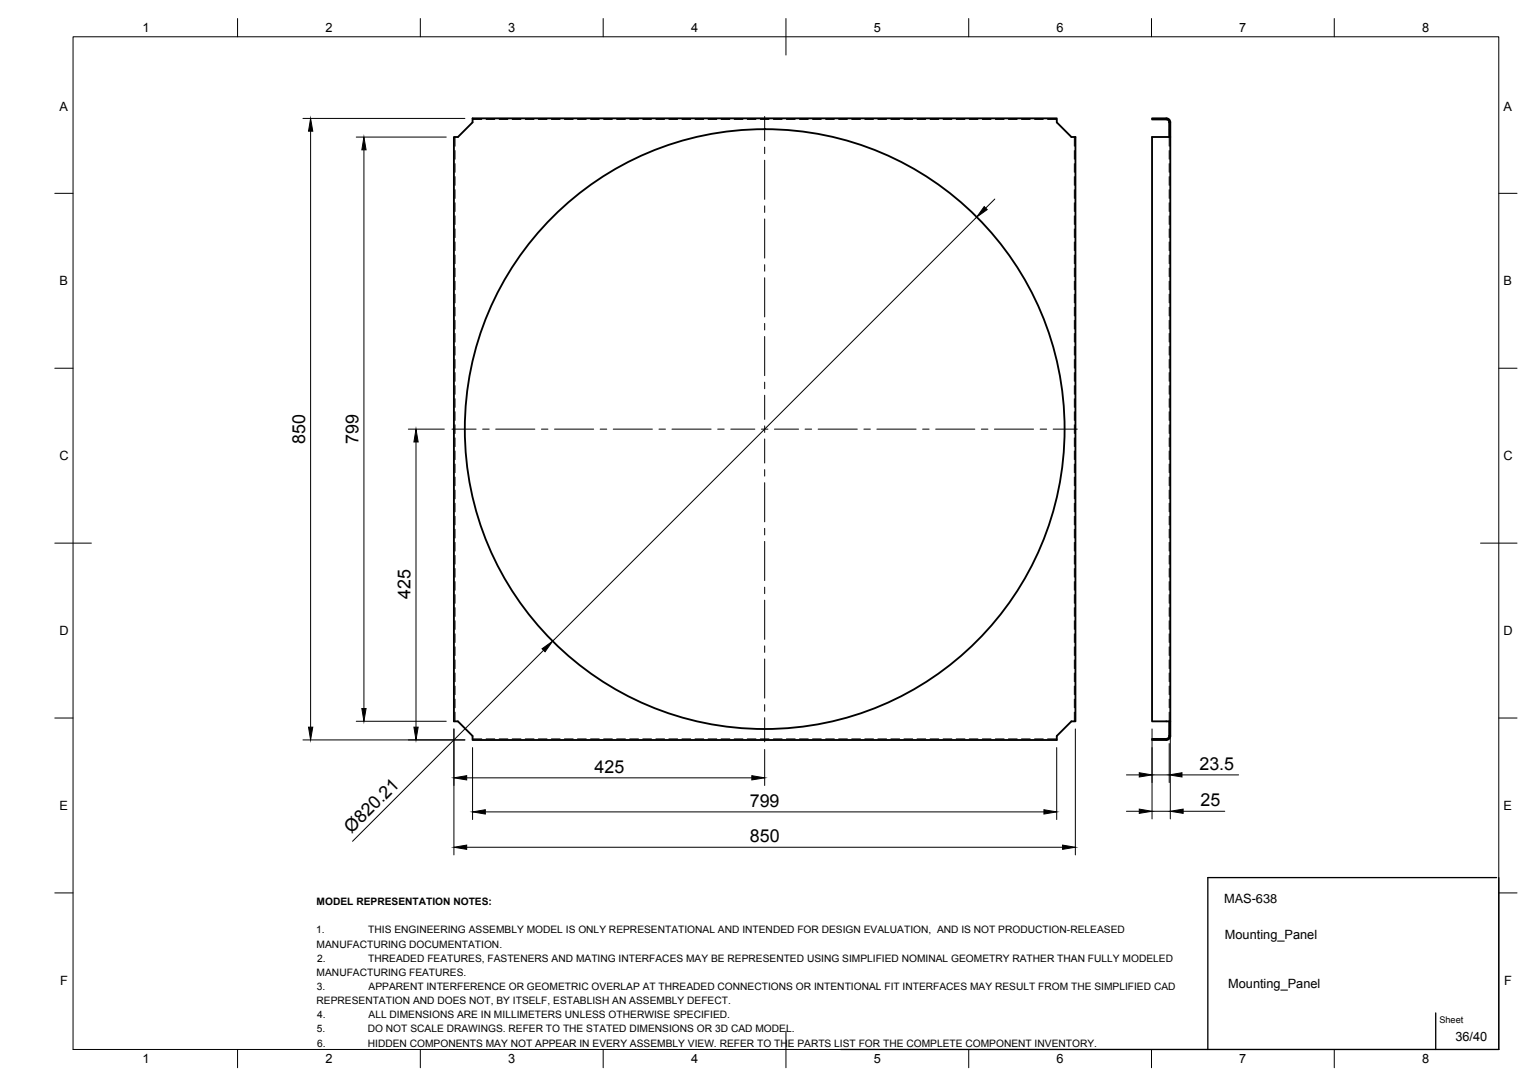
ISO-10303-21;
HEADER;
FILE_DESCRIPTION((''),'2;1');
FILE_NAME('Mounting_Panel.step','2026-10-09T12:00:21-07:00',(''),(''),'','','');
FILE_SCHEMA (('AUTOMOTIVE_DESIGN { 1 0 10303 214 3 1 1 }'));
ENDSEC;
DATA;
#10=MECHANICAL_DESIGN_GEOMETRIC_PRESENTATION_REPRESENTATION('',(#431),#10334);
#151=CYLINDRICAL_SURFACE('',#4171,41.0104872556708) ;
#152=CYLINDRICAL_SURFACE('',#4186,0.549999999999984) ;
#153=CYLINDRICAL_SURFACE('',#4187,0.4) ;
#154=CYLINDRICAL_SURFACE('',#4199,0.549999999999995) ;
#155=CYLINDRICAL_SURFACE('',#4200,0.4) ;
#156=CYLINDRICAL_SURFACE('',#4212,0.549999999999995) ;
#157=CYLINDRICAL_SURFACE('',#4213,0.399999999999995) ;
#158=CYLINDRICAL_SURFACE('',#4225,0.550000000000001) ;
#159=CYLINDRICAL_SURFACE('',#4226,0.4) ;
#359=SHAPE_REPRESENTATION_RELATIONSHIP('SRR','None',#10477,#391) ;
#391=ADVANCED_BREP_SHAPE_REPRESENTATION('',(#463),#10329) ;
#431=STYLED_ITEM('',(#10631),#463) ;
#463=MANIFOLD_SOLID_BREP('Body1',#3585) ;
#475=FACE_BOUND('',#1151,.T.) ;
#476=FACE_BOUND('',#1153,.T.) ;
#498=PLANE('',#4174) ;
#499=PLANE('',#4175) ;
#500=PLANE('',#4176) ;
#501=PLANE('',#4177) ;
#502=PLANE('',#4178) ;
#503=PLANE('',#4179) ;
#504=PLANE('',#4180) ;
#505=PLANE('',#4183) ;
#506=PLANE('',#4188) ;
#507=PLANE('',#4189) ;
#508=PLANE('',#4190) ;
#509=PLANE('',#4191) ;
#510=PLANE('',#4192) ;
#511=PLANE('',#4193) ;
#512=PLANE('',#4196) ;
#513=PLANE('',#4201) ;
#514=PLANE('',#4202) ;
#515=PLANE('',#4203) ;
#516=PLANE('',#4204) ;
#517=PLANE('',#4205) ;
#518=PLANE('',#4206) ;
#519=PLANE('',#4209) ;
#520=PLANE('',#4214) ;
#521=PLANE('',#4215) ;
#522=PLANE('',#4216) ;
#523=PLANE('',#4217) ;
#524=PLANE('',#4218) ;
#525=PLANE('',#4219) ;
#526=PLANE('',#4222) ;
#527=PLANE('',#4227) ;
#528=PLANE('',#4228) ;
#529=PLANE('',#4229) ;
#530=PLANE('',#4230) ;
#531=PLANE('',#4231) ;
#585=LINE('',#9733,#743) ;
#586=LINE('',#9738,#744) ;
#587=LINE('',#9740,#745) ;
#588=LINE('',#9742,#746) ;
#589=LINE('',#9744,#747) ;
#590=LINE('',#9746,#748) ;
#591=LINE('',#9748,#749) ;
#592=LINE('',#9750,#750) ;
#593=LINE('',#9751,#751) ;
#594=LINE('',#9755,#752) ;
#595=LINE('',#9757,#753) ;
#596=LINE('',#9759,#754) ;
#597=LINE('',#9761,#755) ;
#598=LINE('',#9763,#756) ;
#599=LINE('',#9765,#757) ;
#600=LINE('',#9767,#758) ;
#601=LINE('',#9768,#759) ;
#602=LINE('',#9770,#760) ;
#603=LINE('',#9771,#761) ;
#604=LINE('',#9773,#762) ;
#605=LINE('',#9774,#763) ;
#606=LINE('',#9776,#764) ;
#607=LINE('',#9777,#765) ;
#608=LINE('',#9779,#766) ;
#609=LINE('',#9780,#767) ;
#610=LINE('',#9784,#768) ;
#611=LINE('',#9791,#769) ;
#612=LINE('',#9794,#770) ;
#613=LINE('',#9796,#771) ;
#614=LINE('',#9799,#772) ;
#615=LINE('',#9801,#773) ;
#616=LINE('',#9802,#774) ;
#617=LINE('',#9805,#775) ;
#618=LINE('',#9807,#776) ;
#619=LINE('',#9808,#777) ;
#620=LINE('',#9810,#778) ;
#621=LINE('',#9812,#779) ;
#622=LINE('',#9817,#780) ;
#623=LINE('',#9824,#781) ;
#624=LINE('',#9827,#782) ;
#625=LINE('',#9829,#783) ;
#626=LINE('',#9832,#784) ;
#627=LINE('',#9834,#785) ;
#628=LINE('',#9835,#786) ;
#629=LINE('',#9838,#787) ;
#630=LINE('',#9840,#788) ;
#631=LINE('',#9841,#789) ;
#632=LINE('',#9843,#790) ;
#633=LINE('',#9845,#791) ;
#634=LINE('',#9850,#792) ;
#635=LINE('',#9857,#793) ;
#636=LINE('',#9860,#794) ;
#637=LINE('',#9862,#795) ;
#638=LINE('',#9865,#796) ;
#639=LINE('',#9867,#797) ;
#640=LINE('',#9868,#798) ;
#641=LINE('',#9871,#799) ;
#642=LINE('',#9873,#800) ;
#643=LINE('',#9874,#801) ;
#644=LINE('',#9876,#802) ;
#645=LINE('',#9878,#803) ;
#646=LINE('',#9883,#804) ;
#647=LINE('',#9890,#805) ;
#648=LINE('',#9893,#806) ;
#649=LINE('',#9895,#807) ;
#650=LINE('',#9898,#808) ;
#651=LINE('',#9900,#809) ;
#652=LINE('',#9901,#810) ;
#653=LINE('',#9904,#811) ;
#654=LINE('',#9906,#812) ;
#655=LINE('',#9907,#813) ;
#656=LINE('',#9909,#814) ;
#657=LINE('',#9911,#815) ;
#743=VECTOR('',#4957,41.0104872556708) ;
#744=VECTOR('',#4962,100.) ;
#745=VECTOR('',#4963,100.) ;
#746=VECTOR('',#4964,100.) ;
#747=VECTOR('',#4965,100.) ;
#748=VECTOR('',#4966,100.) ;
#749=VECTOR('',#4967,99.9999999999999) ;
#750=VECTOR('',#4968,100.) ;
#751=VECTOR('',#4969,100.) ;
#752=VECTOR('',#4972,100.) ;
#753=VECTOR('',#4973,100.) ;
#754=VECTOR('',#4974,100.) ;
#755=VECTOR('',#4975,100.) ;
#756=VECTOR('',#4976,100.) ;
#757=VECTOR('',#4977,100.) ;
#758=VECTOR('',#4978,100.) ;
#759=VECTOR('',#4979,99.9999999999999) ;
#760=VECTOR('',#4982,100.) ;
#761=VECTOR('',#4983,100.) ;
#762=VECTOR('',#4986,100.) ;
#763=VECTOR('',#4987,100.) ;
#764=VECTOR('',#4990,100.) ;
#765=VECTOR('',#4991,100.) ;
#766=VECTOR('',#4994,100.) ;
#767=VECTOR('',#4995,100.) ;
#768=VECTOR('',#4998,100.) ;
#769=VECTOR('',#5007,100.) ;
#770=VECTOR('',#5012,100.) ;
#771=VECTOR('',#5015,100.) ;
#772=VECTOR('',#5018,100.) ;
#773=VECTOR('',#5019,100.) ;
#774=VECTOR('',#5020,100.) ;
#775=VECTOR('',#5023,100.) ;
#776=VECTOR('',#5024,100.) ;
#777=VECTOR('',#5025,100.) ;
#778=VECTOR('',#5028,100.) ;
#779=VECTOR('',#5031,100.) ;
#780=VECTOR('',#5036,100.) ;
#781=VECTOR('',#5045,100.) ;
#782=VECTOR('',#5050,100.) ;
#783=VECTOR('',#5053,100.) ;
#784=VECTOR('',#5056,100.) ;
#785=VECTOR('',#5057,100.) ;
#786=VECTOR('',#5058,100.) ;
#787=VECTOR('',#5061,100.) ;
#788=VECTOR('',#5062,100.) ;
#789=VECTOR('',#5063,100.) ;
#790=VECTOR('',#5066,100.) ;
#791=VECTOR('',#5069,100.) ;
#792=VECTOR('',#5074,100.) ;
#793=VECTOR('',#5083,100.) ;
#794=VECTOR('',#5088,100.) ;
#795=VECTOR('',#5091,100.) ;
#796=VECTOR('',#5094,100.) ;
#797=VECTOR('',#5095,100.) ;
#798=VECTOR('',#5096,100.) ;
#799=VECTOR('',#5099,100.) ;
#800=VECTOR('',#5100,100.) ;
#801=VECTOR('',#5101,100.) ;
#802=VECTOR('',#5104,100.) ;
#803=VECTOR('',#5107,100.) ;
#804=VECTOR('',#5112,100.) ;
#805=VECTOR('',#5121,100.) ;
#806=VECTOR('',#5126,100.) ;
#807=VECTOR('',#5129,100.) ;
#808=VECTOR('',#5132,100.) ;
#809=VECTOR('',#5133,100.) ;
#810=VECTOR('',#5134,100.) ;
#811=VECTOR('',#5137,100.) ;
#812=VECTOR('',#5138,100.) ;
#813=VECTOR('',#5139,100.) ;
#814=VECTOR('',#5142,100.) ;
#815=VECTOR('',#5145,100.) ;
#943=FACE_OUTER_BOUND('',#1149,.T.) ;
#944=FACE_OUTER_BOUND('',#1150,.T.) ;
#945=FACE_OUTER_BOUND('',#1152,.T.) ;
#946=FACE_OUTER_BOUND('',#1154,.T.) ;
#947=FACE_OUTER_BOUND('',#1155,.T.) ;
#948=FACE_OUTER_BOUND('',#1156,.T.) ;
#949=FACE_OUTER_BOUND('',#1157,.T.) ;
#950=FACE_OUTER_BOUND('',#1158,.T.) ;
#951=FACE_OUTER_BOUND('',#1159,.T.) ;
#952=FACE_OUTER_BOUND('',#1160,.T.) ;
#953=FACE_OUTER_BOUND('',#1161,.T.) ;
#954=FACE_OUTER_BOUND('',#1162,.T.) ;
#955=FACE_OUTER_BOUND('',#1163,.T.) ;
#956=FACE_OUTER_BOUND('',#1164,.T.) ;
#957=FACE_OUTER_BOUND('',#1165,.T.) ;
#958=FACE_OUTER_BOUND('',#1166,.T.) ;
#959=FACE_OUTER_BOUND('',#1167,.T.) ;
#960=FACE_OUTER_BOUND('',#1168,.T.) ;
#961=FACE_OUTER_BOUND('',#1169,.T.) ;
#962=FACE_OUTER_BOUND('',#1170,.T.) ;
#963=FACE_OUTER_BOUND('',#1171,.T.) ;
#964=FACE_OUTER_BOUND('',#1172,.T.) ;
#965=FACE_OUTER_BOUND('',#1173,.T.) ;
#966=FACE_OUTER_BOUND('',#1174,.T.) ;
#967=FACE_OUTER_BOUND('',#1175,.T.) ;
#968=FACE_OUTER_BOUND('',#1176,.T.) ;
#969=FACE_OUTER_BOUND('',#1177,.T.) ;
#970=FACE_OUTER_BOUND('',#1178,.T.) ;
#971=FACE_OUTER_BOUND('',#1179,.T.) ;
#972=FACE_OUTER_BOUND('',#1180,.T.) ;
#973=FACE_OUTER_BOUND('',#1181,.T.) ;
#974=FACE_OUTER_BOUND('',#1182,.T.) ;
#975=FACE_OUTER_BOUND('',#1183,.T.) ;
#976=FACE_OUTER_BOUND('',#1184,.T.) ;
#977=FACE_OUTER_BOUND('',#1185,.T.) ;
#978=FACE_OUTER_BOUND('',#1186,.T.) ;
#979=FACE_OUTER_BOUND('',#1187,.T.) ;
#980=FACE_OUTER_BOUND('',#1188,.T.) ;
#981=FACE_OUTER_BOUND('',#1189,.T.) ;
#982=FACE_OUTER_BOUND('',#1190,.T.) ;
#983=FACE_OUTER_BOUND('',#1191,.T.) ;
#984=FACE_OUTER_BOUND('',#1192,.T.) ;
#985=FACE_OUTER_BOUND('',#1193,.T.) ;
#1149=EDGE_LOOP('',(#2783,#2784,#2785,#2786)) ;
#1150=EDGE_LOOP('',(#2787,#2788,#2789,#2790,#2791,#2792,#2793,#2794)) ;
#1151=EDGE_LOOP('',(#2795)) ;
#1152=EDGE_LOOP('',(#2796,#2797,#2798,#2799,#2800,#2801,#2802,#2803)) ;
#1153=EDGE_LOOP('',(#2804)) ;
#1154=EDGE_LOOP('',(#2805,#2806,#2807,#2808)) ;
#1155=EDGE_LOOP('',(#2809,#2810,#2811,#2812)) ;
#1156=EDGE_LOOP('',(#2813,#2814,#2815,#2816)) ;
#1157=EDGE_LOOP('',(#2817,#2818,#2819,#2820)) ;
#1158=EDGE_LOOP('',(#2821,#2822,#2823,#2824)) ;
#1159=EDGE_LOOP('',(#2825,#2826,#2827,#2828)) ;
#1160=EDGE_LOOP('',(#2829,#2830,#2831,#2832)) ;
#1161=EDGE_LOOP('',(#2833,#2834,#2835,#2836)) ;
#1162=EDGE_LOOP('',(#2837,#2838,#2839,#2840)) ;
#1163=EDGE_LOOP('',(#2841,#2842,#2843,#2844)) ;
#1164=EDGE_LOOP('',(#2845,#2846,#2847,#2848)) ;
#1165=EDGE_LOOP('',(#2849,#2850,#2851,#2852)) ;
#1166=EDGE_LOOP('',(#2853,#2854,#2855,#2856)) ;
#1167=EDGE_LOOP('',(#2857,#2858,#2859,#2860)) ;
#1168=EDGE_LOOP('',(#2861,#2862,#2863,#2864)) ;
#1169=EDGE_LOOP('',(#2865,#2866,#2867,#2868)) ;
#1170=EDGE_LOOP('',(#2869,#2870,#2871,#2872)) ;
#1171=EDGE_LOOP('',(#2873,#2874,#2875,#2876)) ;
#1172=EDGE_LOOP('',(#2877,#2878,#2879,#2880)) ;
#1173=EDGE_LOOP('',(#2881,#2882,#2883,#2884)) ;
#1174=EDGE_LOOP('',(#2885,#2886,#2887,#2888)) ;
#1175=EDGE_LOOP('',(#2889,#2890,#2891,#2892)) ;
#1176=EDGE_LOOP('',(#2893,#2894,#2895,#2896)) ;
#1177=EDGE_LOOP('',(#2897,#2898,#2899,#2900)) ;
#1178=EDGE_LOOP('',(#2901,#2902,#2903,#2904)) ;
#1179=EDGE_LOOP('',(#2905,#2906,#2907,#2908)) ;
#1180=EDGE_LOOP('',(#2909,#2910,#2911,#2912)) ;
#1181=EDGE_LOOP('',(#2913,#2914,#2915,#2916)) ;
#1182=EDGE_LOOP('',(#2917,#2918,#2919,#2920)) ;
#1183=EDGE_LOOP('',(#2921,#2922,#2923,#2924)) ;
#1184=EDGE_LOOP('',(#2925,#2926,#2927,#2928)) ;
#1185=EDGE_LOOP('',(#2929,#2930,#2931,#2932)) ;
#1186=EDGE_LOOP('',(#2933,#2934,#2935,#2936)) ;
#1187=EDGE_LOOP('',(#2937,#2938,#2939,#2940)) ;
#1188=EDGE_LOOP('',(#2941,#2942,#2943,#2944)) ;
#1189=EDGE_LOOP('',(#2945,#2946,#2947,#2948)) ;
#1190=EDGE_LOOP('',(#2949,#2950,#2951,#2952)) ;
#1191=EDGE_LOOP('',(#2953,#2954,#2955,#2956)) ;
#1192=EDGE_LOOP('',(#2957,#2958,#2959,#2960)) ;
#1193=EDGE_LOOP('',(#2961,#2962,#2963,#2964)) ;
#1345=CIRCLE('',#4172,41.0104872556708) ;
#1346=CIRCLE('',#4173,41.0104872556708) ;
#1347=CIRCLE('',#4181,0.399999999999995) ;
#1348=CIRCLE('',#4182,0.549999999999995) ;
#1349=CIRCLE('',#4184,0.399999999999995) ;
#1350=CIRCLE('',#4185,0.549999999999995) ;
#1351=CIRCLE('',#4194,0.4) ;
#1352=CIRCLE('',#4195,0.550000000000001) ;
#1353=CIRCLE('',#4197,0.4) ;
#1354=CIRCLE('',#4198,0.550000000000001) ;
#1355=CIRCLE('',#4207,0.399999999999995) ;
#1356=CIRCLE('',#4208,0.549999999999995) ;
#1357=CIRCLE('',#4210,0.399999999999995) ;
#1358=CIRCLE('',#4211,0.549999999999995) ;
#1359=CIRCLE('',#4220,0.4) ;
#1360=CIRCLE('',#4221,0.550000000000001) ;
#1361=CIRCLE('',#4223,0.4) ;
#1362=CIRCLE('',#4224,0.550000000000001) ;
#1656=VERTEX_POINT('',#9730) ;
#1657=VERTEX_POINT('',#9732) ;
#1658=VERTEX_POINT('',#9736) ;
#1659=VERTEX_POINT('',#9737) ;
#1660=VERTEX_POINT('',#9739) ;
#1661=VERTEX_POINT('',#9741) ;
#1662=VERTEX_POINT('',#9743) ;
#1663=VERTEX_POINT('',#9745) ;
#1664=VERTEX_POINT('',#9747) ;
#1665=VERTEX_POINT('',#9749) ;
#1666=VERTEX_POINT('',#9753) ;
#1667=VERTEX_POINT('',#9754) ;
#1668=VERTEX_POINT('',#9756) ;
#1669=VERTEX_POINT('',#9758) ;
#1670=VERTEX_POINT('',#9760) ;
#1671=VERTEX_POINT('',#9762) ;
#1672=VERTEX_POINT('',#9764) ;
#1673=VERTEX_POINT('',#9766) ;
#1674=VERTEX_POINT('',#9782) ;
#1675=VERTEX_POINT('',#9783) ;
#1676=VERTEX_POINT('',#9788) ;
#1677=VERTEX_POINT('',#9790) ;
#1678=VERTEX_POINT('',#9798) ;
#1679=VERTEX_POINT('',#9800) ;
#1680=VERTEX_POINT('',#9804) ;
#1681=VERTEX_POINT('',#9806) ;
#1682=VERTEX_POINT('',#9815) ;
#1683=VERTEX_POINT('',#9816) ;
#1684=VERTEX_POINT('',#9821) ;
#1685=VERTEX_POINT('',#9823) ;
#1686=VERTEX_POINT('',#9831) ;
#1687=VERTEX_POINT('',#9833) ;
#1688=VERTEX_POINT('',#9837) ;
#1689=VERTEX_POINT('',#9839) ;
#1690=VERTEX_POINT('',#9848) ;
#1691=VERTEX_POINT('',#9849) ;
#1692=VERTEX_POINT('',#9854) ;
#1693=VERTEX_POINT('',#9856) ;
#1694=VERTEX_POINT('',#9864) ;
#1695=VERTEX_POINT('',#9866) ;
#1696=VERTEX_POINT('',#9870) ;
#1697=VERTEX_POINT('',#9872) ;
#1698=VERTEX_POINT('',#9881) ;
#1699=VERTEX_POINT('',#9882) ;
#1700=VERTEX_POINT('',#9887) ;
#1701=VERTEX_POINT('',#9889) ;
#1702=VERTEX_POINT('',#9897) ;
#1703=VERTEX_POINT('',#9899) ;
#1704=VERTEX_POINT('',#9903) ;
#1705=VERTEX_POINT('',#9905) ;
#2048=EDGE_CURVE('',#1656,#1656,#1345,.T.) ;
#2049=EDGE_CURVE('',#1656,#1657,#585,.T.) ;
#2050=EDGE_CURVE('',#1657,#1657,#1346,.T.) ;
#2051=EDGE_CURVE('',#1658,#1659,#586,.T.) ;
#2052=EDGE_CURVE('',#1658,#1660,#587,.T.) ;
#2053=EDGE_CURVE('',#1661,#1660,#588,.T.) ;
#2054=EDGE_CURVE('',#1661,#1662,#589,.T.) ;
#2055=EDGE_CURVE('',#1663,#1662,#590,.T.) ;
#2056=EDGE_CURVE('',#1663,#1664,#591,.T.) ;
#2057=EDGE_CURVE('',#1665,#1664,#592,.T.) ;
#2058=EDGE_CURVE('',#1665,#1659,#593,.T.) ;
#2059=EDGE_CURVE('',#1666,#1667,#594,.T.) ;
#2060=EDGE_CURVE('',#1667,#1668,#595,.T.) ;
#2061=EDGE_CURVE('',#1668,#1669,#596,.T.) ;
#2062=EDGE_CURVE('',#1669,#1670,#597,.T.) ;
#2063=EDGE_CURVE('',#1670,#1671,#598,.T.) ;
#2064=EDGE_CURVE('',#1671,#1672,#599,.T.) ;
#2065=EDGE_CURVE('',#1672,#1673,#600,.T.) ;
#2066=EDGE_CURVE('',#1673,#1666,#601,.T.) ;
#2067=EDGE_CURVE('',#1668,#1658,#602,.T.) ;
#2068=EDGE_CURVE('',#1660,#1667,#603,.T.) ;
#2069=EDGE_CURVE('',#1666,#1661,#604,.T.) ;
#2070=EDGE_CURVE('',#1662,#1673,#605,.T.) ;
#2071=EDGE_CURVE('',#1672,#1663,#606,.T.) ;
#2072=EDGE_CURVE('',#1664,#1671,#607,.T.) ;
#2073=EDGE_CURVE('',#1670,#1665,#608,.T.) ;
#2074=EDGE_CURVE('',#1659,#1669,#609,.T.) ;
#2075=EDGE_CURVE('',#1674,#1675,#610,.T.) ;
#2076=EDGE_CURVE('',#1664,#1674,#1347,.T.) ;
#2077=EDGE_CURVE('',#1671,#1675,#1348,.T.) ;
#2078=EDGE_CURVE('',#1676,#1665,#1349,.T.) ;
#2079=EDGE_CURVE('',#1676,#1677,#611,.T.) ;
#2080=EDGE_CURVE('',#1677,#1670,#1350,.T.) ;
#2081=EDGE_CURVE('',#1677,#1675,#612,.T.) ;
#2082=EDGE_CURVE('',#1674,#1676,#613,.T.) ;
#2083=EDGE_CURVE('',#1676,#1678,#614,.T.) ;
#2084=EDGE_CURVE('',#1679,#1678,#615,.T.) ;
#2085=EDGE_CURVE('',#1677,#1679,#616,.T.) ;
#2086=EDGE_CURVE('',#1680,#1675,#617,.T.) ;
#2087=EDGE_CURVE('',#1680,#1681,#618,.T.) ;
#2088=EDGE_CURVE('',#1681,#1674,#619,.T.) ;
#2089=EDGE_CURVE('',#1679,#1680,#620,.T.) ;
#2090=EDGE_CURVE('',#1678,#1681,#621,.T.) ;
#2091=EDGE_CURVE('',#1682,#1683,#622,.T.) ;
#2092=EDGE_CURVE('',#1659,#1682,#1351,.T.) ;
#2093=EDGE_CURVE('',#1669,#1683,#1352,.T.) ;
#2094=EDGE_CURVE('',#1684,#1658,#1353,.T.) ;
#2095=EDGE_CURVE('',#1684,#1685,#623,.T.) ;
#2096=EDGE_CURVE('',#1685,#1668,#1354,.T.) ;
#2097=EDGE_CURVE('',#1685,#1683,#624,.T.) ;
#2098=EDGE_CURVE('',#1682,#1684,#625,.T.) ;
#2099=EDGE_CURVE('',#1684,#1686,#626,.T.) ;
#2100=EDGE_CURVE('',#1687,#1686,#627,.T.) ;
#2101=EDGE_CURVE('',#1685,#1687,#628,.T.) ;
#2102=EDGE_CURVE('',#1688,#1683,#629,.T.) ;
#2103=EDGE_CURVE('',#1688,#1689,#630,.T.) ;
#2104=EDGE_CURVE('',#1689,#1682,#631,.T.) ;
#2105=EDGE_CURVE('',#1687,#1688,#632,.T.) ;
#2106=EDGE_CURVE('',#1686,#1689,#633,.T.) ;
#2107=EDGE_CURVE('',#1690,#1691,#634,.T.) ;
#2108=EDGE_CURVE('',#1660,#1690,#1355,.T.) ;
#2109=EDGE_CURVE('',#1667,#1691,#1356,.T.) ;
#2110=EDGE_CURVE('',#1692,#1661,#1357,.T.) ;
#2111=EDGE_CURVE('',#1692,#1693,#635,.T.) ;
#2112=EDGE_CURVE('',#1693,#1666,#1358,.T.) ;
#2113=EDGE_CURVE('',#1693,#1691,#636,.T.) ;
#2114=EDGE_CURVE('',#1690,#1692,#637,.T.) ;
#2115=EDGE_CURVE('',#1692,#1694,#638,.T.) ;
#2116=EDGE_CURVE('',#1695,#1694,#639,.T.) ;
#2117=EDGE_CURVE('',#1693,#1695,#640,.T.) ;
#2118=EDGE_CURVE('',#1696,#1691,#641,.T.) ;
#2119=EDGE_CURVE('',#1696,#1697,#642,.T.) ;
#2120=EDGE_CURVE('',#1697,#1690,#643,.T.) ;
#2121=EDGE_CURVE('',#1695,#1696,#644,.T.) ;
#2122=EDGE_CURVE('',#1694,#1697,#645,.T.) ;
#2123=EDGE_CURVE('',#1698,#1699,#646,.T.) ;
#2124=EDGE_CURVE('',#1662,#1698,#1359,.T.) ;
#2125=EDGE_CURVE('',#1673,#1699,#1360,.T.) ;
#2126=EDGE_CURVE('',#1700,#1663,#1361,.T.) ;
#2127=EDGE_CURVE('',#1700,#1701,#647,.T.) ;
#2128=EDGE_CURVE('',#1701,#1672,#1362,.T.) ;
#2129=EDGE_CURVE('',#1701,#1699,#648,.T.) ;
#2130=EDGE_CURVE('',#1698,#1700,#649,.T.) ;
#2131=EDGE_CURVE('',#1700,#1702,#650,.T.) ;
#2132=EDGE_CURVE('',#1703,#1702,#651,.T.) ;
#2133=EDGE_CURVE('',#1701,#1703,#652,.T.) ;
#2134=EDGE_CURVE('',#1704,#1699,#653,.T.) ;
#2135=EDGE_CURVE('',#1704,#1705,#654,.T.) ;
#2136=EDGE_CURVE('',#1705,#1698,#655,.T.) ;
#2137=EDGE_CURVE('',#1703,#1704,#656,.T.) ;
#2138=EDGE_CURVE('',#1702,#1705,#657,.T.) ;
#2783=ORIENTED_EDGE('',*,*,#2048,.F.) ;
#2784=ORIENTED_EDGE('',*,*,#2049,.T.) ;
#2785=ORIENTED_EDGE('',*,*,#2050,.T.) ;
#2786=ORIENTED_EDGE('',*,*,#2049,.F.) ;
#2787=ORIENTED_EDGE('',*,*,#2051,.F.) ;
#2788=ORIENTED_EDGE('',*,*,#2052,.T.) ;
#2789=ORIENTED_EDGE('',*,*,#2053,.F.) ;
#2790=ORIENTED_EDGE('',*,*,#2054,.T.) ;
#2791=ORIENTED_EDGE('',*,*,#2055,.F.) ;
#2792=ORIENTED_EDGE('',*,*,#2056,.T.) ;
#2793=ORIENTED_EDGE('',*,*,#2057,.F.) ;
#2794=ORIENTED_EDGE('',*,*,#2058,.T.) ;
#2795=ORIENTED_EDGE('',*,*,#2048,.T.) ;
#2796=ORIENTED_EDGE('',*,*,#2059,.T.) ;
#2797=ORIENTED_EDGE('',*,*,#2060,.T.) ;
#2798=ORIENTED_EDGE('',*,*,#2061,.T.) ;
#2799=ORIENTED_EDGE('',*,*,#2062,.T.) ;
#2800=ORIENTED_EDGE('',*,*,#2063,.T.) ;
#2801=ORIENTED_EDGE('',*,*,#2064,.T.) ;
#2802=ORIENTED_EDGE('',*,*,#2065,.T.) ;
#2803=ORIENTED_EDGE('',*,*,#2066,.T.) ;
#2804=ORIENTED_EDGE('',*,*,#2050,.F.) ;
#2805=ORIENTED_EDGE('',*,*,#2052,.F.) ;
#2806=ORIENTED_EDGE('',*,*,#2067,.F.) ;
#2807=ORIENTED_EDGE('',*,*,#2060,.F.) ;
#2808=ORIENTED_EDGE('',*,*,#2068,.F.) ;
#2809=ORIENTED_EDGE('',*,*,#2054,.F.) ;
#2810=ORIENTED_EDGE('',*,*,#2069,.F.) ;
#2811=ORIENTED_EDGE('',*,*,#2066,.F.) ;
#2812=ORIENTED_EDGE('',*,*,#2070,.F.) ;
#2813=ORIENTED_EDGE('',*,*,#2056,.F.) ;
#2814=ORIENTED_EDGE('',*,*,#2071,.F.) ;
#2815=ORIENTED_EDGE('',*,*,#2064,.F.) ;
#2816=ORIENTED_EDGE('',*,*,#2072,.F.) ;
#2817=ORIENTED_EDGE('',*,*,#2058,.F.) ;
#2818=ORIENTED_EDGE('',*,*,#2073,.F.) ;
#2819=ORIENTED_EDGE('',*,*,#2062,.F.) ;
#2820=ORIENTED_EDGE('',*,*,#2074,.F.) ;
#2821=ORIENTED_EDGE('',*,*,#2075,.F.) ;
#2822=ORIENTED_EDGE('',*,*,#2076,.F.) ;
#2823=ORIENTED_EDGE('',*,*,#2072,.T.) ;
#2824=ORIENTED_EDGE('',*,*,#2077,.T.) ;
#2825=ORIENTED_EDGE('',*,*,#2078,.F.) ;
#2826=ORIENTED_EDGE('',*,*,#2079,.T.) ;
#2827=ORIENTED_EDGE('',*,*,#2080,.T.) ;
#2828=ORIENTED_EDGE('',*,*,#2073,.T.) ;
#2829=ORIENTED_EDGE('',*,*,#2063,.F.) ;
#2830=ORIENTED_EDGE('',*,*,#2080,.F.) ;
#2831=ORIENTED_EDGE('',*,*,#2081,.T.) ;
#2832=ORIENTED_EDGE('',*,*,#2077,.F.) ;
#2833=ORIENTED_EDGE('',*,*,#2057,.T.) ;
#2834=ORIENTED_EDGE('',*,*,#2076,.T.) ;
#2835=ORIENTED_EDGE('',*,*,#2082,.T.) ;
#2836=ORIENTED_EDGE('',*,*,#2078,.T.) ;
#2837=ORIENTED_EDGE('',*,*,#2079,.F.) ;
#2838=ORIENTED_EDGE('',*,*,#2083,.T.) ;
#2839=ORIENTED_EDGE('',*,*,#2084,.F.) ;
#2840=ORIENTED_EDGE('',*,*,#2085,.F.) ;
#2841=ORIENTED_EDGE('',*,*,#2075,.T.) ;
#2842=ORIENTED_EDGE('',*,*,#2086,.F.) ;
#2843=ORIENTED_EDGE('',*,*,#2087,.T.) ;
#2844=ORIENTED_EDGE('',*,*,#2088,.T.) ;
#2845=ORIENTED_EDGE('',*,*,#2081,.F.) ;
#2846=ORIENTED_EDGE('',*,*,#2085,.T.) ;
#2847=ORIENTED_EDGE('',*,*,#2089,.T.) ;
#2848=ORIENTED_EDGE('',*,*,#2086,.T.) ;
#2849=ORIENTED_EDGE('',*,*,#2083,.F.) ;
#2850=ORIENTED_EDGE('',*,*,#2082,.F.) ;
#2851=ORIENTED_EDGE('',*,*,#2088,.F.) ;
#2852=ORIENTED_EDGE('',*,*,#2090,.F.) ;
#2853=ORIENTED_EDGE('',*,*,#2090,.T.) ;
#2854=ORIENTED_EDGE('',*,*,#2087,.F.) ;
#2855=ORIENTED_EDGE('',*,*,#2089,.F.) ;
#2856=ORIENTED_EDGE('',*,*,#2084,.T.) ;
#2857=ORIENTED_EDGE('',*,*,#2091,.F.) ;
#2858=ORIENTED_EDGE('',*,*,#2092,.F.) ;
#2859=ORIENTED_EDGE('',*,*,#2074,.T.) ;
#2860=ORIENTED_EDGE('',*,*,#2093,.T.) ;
#2861=ORIENTED_EDGE('',*,*,#2094,.F.) ;
#2862=ORIENTED_EDGE('',*,*,#2095,.T.) ;
#2863=ORIENTED_EDGE('',*,*,#2096,.T.) ;
#2864=ORIENTED_EDGE('',*,*,#2067,.T.) ;
#2865=ORIENTED_EDGE('',*,*,#2061,.F.) ;
#2866=ORIENTED_EDGE('',*,*,#2096,.F.) ;
#2867=ORIENTED_EDGE('',*,*,#2097,.T.) ;
#2868=ORIENTED_EDGE('',*,*,#2093,.F.) ;
#2869=ORIENTED_EDGE('',*,*,#2051,.T.) ;
#2870=ORIENTED_EDGE('',*,*,#2092,.T.) ;
#2871=ORIENTED_EDGE('',*,*,#2098,.T.) ;
#2872=ORIENTED_EDGE('',*,*,#2094,.T.) ;
#2873=ORIENTED_EDGE('',*,*,#2095,.F.) ;
#2874=ORIENTED_EDGE('',*,*,#2099,.T.) ;
#2875=ORIENTED_EDGE('',*,*,#2100,.F.) ;
#2876=ORIENTED_EDGE('',*,*,#2101,.F.) ;
#2877=ORIENTED_EDGE('',*,*,#2091,.T.) ;
#2878=ORIENTED_EDGE('',*,*,#2102,.F.) ;
#2879=ORIENTED_EDGE('',*,*,#2103,.T.) ;
#2880=ORIENTED_EDGE('',*,*,#2104,.T.) ;
#2881=ORIENTED_EDGE('',*,*,#2097,.F.) ;
#2882=ORIENTED_EDGE('',*,*,#2101,.T.) ;
#2883=ORIENTED_EDGE('',*,*,#2105,.T.) ;
#2884=ORIENTED_EDGE('',*,*,#2102,.T.) ;
#2885=ORIENTED_EDGE('',*,*,#2099,.F.) ;
#2886=ORIENTED_EDGE('',*,*,#2098,.F.) ;
#2887=ORIENTED_EDGE('',*,*,#2104,.F.) ;
#2888=ORIENTED_EDGE('',*,*,#2106,.F.) ;
#2889=ORIENTED_EDGE('',*,*,#2106,.T.) ;
#2890=ORIENTED_EDGE('',*,*,#2103,.F.) ;
#2891=ORIENTED_EDGE('',*,*,#2105,.F.) ;
#2892=ORIENTED_EDGE('',*,*,#2100,.T.) ;
#2893=ORIENTED_EDGE('',*,*,#2107,.F.) ;
#2894=ORIENTED_EDGE('',*,*,#2108,.F.) ;
#2895=ORIENTED_EDGE('',*,*,#2068,.T.) ;
#2896=ORIENTED_EDGE('',*,*,#2109,.T.) ;
#2897=ORIENTED_EDGE('',*,*,#2110,.F.) ;
#2898=ORIENTED_EDGE('',*,*,#2111,.T.) ;
#2899=ORIENTED_EDGE('',*,*,#2112,.T.) ;
#2900=ORIENTED_EDGE('',*,*,#2069,.T.) ;
#2901=ORIENTED_EDGE('',*,*,#2059,.F.) ;
#2902=ORIENTED_EDGE('',*,*,#2112,.F.) ;
#2903=ORIENTED_EDGE('',*,*,#2113,.T.) ;
#2904=ORIENTED_EDGE('',*,*,#2109,.F.) ;
#2905=ORIENTED_EDGE('',*,*,#2053,.T.) ;
#2906=ORIENTED_EDGE('',*,*,#2108,.T.) ;
#2907=ORIENTED_EDGE('',*,*,#2114,.T.) ;
#2908=ORIENTED_EDGE('',*,*,#2110,.T.) ;
#2909=ORIENTED_EDGE('',*,*,#2111,.F.) ;
#2910=ORIENTED_EDGE('',*,*,#2115,.T.) ;
#2911=ORIENTED_EDGE('',*,*,#2116,.F.) ;
#2912=ORIENTED_EDGE('',*,*,#2117,.F.) ;
#2913=ORIENTED_EDGE('',*,*,#2107,.T.) ;
#2914=ORIENTED_EDGE('',*,*,#2118,.F.) ;
#2915=ORIENTED_EDGE('',*,*,#2119,.T.) ;
#2916=ORIENTED_EDGE('',*,*,#2120,.T.) ;
#2917=ORIENTED_EDGE('',*,*,#2113,.F.) ;
#2918=ORIENTED_EDGE('',*,*,#2117,.T.) ;
#2919=ORIENTED_EDGE('',*,*,#2121,.T.) ;
#2920=ORIENTED_EDGE('',*,*,#2118,.T.) ;
#2921=ORIENTED_EDGE('',*,*,#2115,.F.) ;
#2922=ORIENTED_EDGE('',*,*,#2114,.F.) ;
#2923=ORIENTED_EDGE('',*,*,#2120,.F.) ;
#2924=ORIENTED_EDGE('',*,*,#2122,.F.) ;
#2925=ORIENTED_EDGE('',*,*,#2122,.T.) ;
#2926=ORIENTED_EDGE('',*,*,#2119,.F.) ;
#2927=ORIENTED_EDGE('',*,*,#2121,.F.) ;
#2928=ORIENTED_EDGE('',*,*,#2116,.T.) ;
#2929=ORIENTED_EDGE('',*,*,#2123,.F.) ;
#2930=ORIENTED_EDGE('',*,*,#2124,.F.) ;
#2931=ORIENTED_EDGE('',*,*,#2070,.T.) ;
#2932=ORIENTED_EDGE('',*,*,#2125,.T.) ;
#2933=ORIENTED_EDGE('',*,*,#2126,.F.) ;
#2934=ORIENTED_EDGE('',*,*,#2127,.T.) ;
#2935=ORIENTED_EDGE('',*,*,#2128,.T.) ;
#2936=ORIENTED_EDGE('',*,*,#2071,.T.) ;
#2937=ORIENTED_EDGE('',*,*,#2065,.F.) ;
#2938=ORIENTED_EDGE('',*,*,#2128,.F.) ;
#2939=ORIENTED_EDGE('',*,*,#2129,.T.) ;
#2940=ORIENTED_EDGE('',*,*,#2125,.F.) ;
#2941=ORIENTED_EDGE('',*,*,#2055,.T.) ;
#2942=ORIENTED_EDGE('',*,*,#2124,.T.) ;
#2943=ORIENTED_EDGE('',*,*,#2130,.T.) ;
#2944=ORIENTED_EDGE('',*,*,#2126,.T.) ;
#2945=ORIENTED_EDGE('',*,*,#2127,.F.) ;
#2946=ORIENTED_EDGE('',*,*,#2131,.T.) ;
#2947=ORIENTED_EDGE('',*,*,#2132,.F.) ;
#2948=ORIENTED_EDGE('',*,*,#2133,.F.) ;
#2949=ORIENTED_EDGE('',*,*,#2123,.T.) ;
#2950=ORIENTED_EDGE('',*,*,#2134,.F.) ;
#2951=ORIENTED_EDGE('',*,*,#2135,.T.) ;
#2952=ORIENTED_EDGE('',*,*,#2136,.T.) ;
#2953=ORIENTED_EDGE('',*,*,#2129,.F.) ;
#2954=ORIENTED_EDGE('',*,*,#2133,.T.) ;
#2955=ORIENTED_EDGE('',*,*,#2137,.T.) ;
#2956=ORIENTED_EDGE('',*,*,#2134,.T.) ;
#2957=ORIENTED_EDGE('',*,*,#2131,.F.) ;
#2958=ORIENTED_EDGE('',*,*,#2130,.F.) ;
#2959=ORIENTED_EDGE('',*,*,#2136,.F.) ;
#2960=ORIENTED_EDGE('',*,*,#2138,.F.) ;
#2961=ORIENTED_EDGE('',*,*,#2138,.T.) ;
#2962=ORIENTED_EDGE('',*,*,#2135,.F.) ;
#2963=ORIENTED_EDGE('',*,*,#2137,.F.) ;
#2964=ORIENTED_EDGE('',*,*,#2132,.T.) ;
#3451=ADVANCED_FACE('',(#943),#151,.F.) ;
#3452=ADVANCED_FACE('',(#944,#475),#498,.F.) ;
#3453=ADVANCED_FACE('',(#945,#476),#499,.T.) ;
#3454=ADVANCED_FACE('',(#946),#500,.F.) ;
#3455=ADVANCED_FACE('',(#947),#501,.F.) ;
#3456=ADVANCED_FACE('',(#948),#502,.F.) ;
#3457=ADVANCED_FACE('',(#949),#503,.F.) ;
#3458=ADVANCED_FACE('',(#950),#504,.T.) ;
#3459=ADVANCED_FACE('',(#951),#505,.F.) ;
#3460=ADVANCED_FACE('',(#952),#152,.T.) ;
#3461=ADVANCED_FACE('',(#953),#153,.F.) ;
#3462=ADVANCED_FACE('',(#954),#506,.F.) ;
#3463=ADVANCED_FACE('',(#955),#507,.F.) ;
#3464=ADVANCED_FACE('',(#956),#508,.F.) ;
#3465=ADVANCED_FACE('',(#957),#509,.T.) ;
#3466=ADVANCED_FACE('',(#958),#510,.F.) ;
#3467=ADVANCED_FACE('',(#959),#511,.T.) ;
#3468=ADVANCED_FACE('',(#960),#512,.F.) ;
#3469=ADVANCED_FACE('',(#961),#154,.T.) ;
#3470=ADVANCED_FACE('',(#962),#155,.F.) ;
#3471=ADVANCED_FACE('',(#963),#513,.F.) ;
#3472=ADVANCED_FACE('',(#964),#514,.F.) ;
#3473=ADVANCED_FACE('',(#965),#515,.F.) ;
#3474=ADVANCED_FACE('',(#966),#516,.T.) ;
#3475=ADVANCED_FACE('',(#967),#517,.F.) ;
#3476=ADVANCED_FACE('',(#968),#518,.T.) ;
#3477=ADVANCED_FACE('',(#969),#519,.F.) ;
#3478=ADVANCED_FACE('',(#970),#156,.T.) ;
#3479=ADVANCED_FACE('',(#971),#157,.F.) ;
#3480=ADVANCED_FACE('',(#972),#520,.F.) ;
#3481=ADVANCED_FACE('',(#973),#521,.F.) ;
#3482=ADVANCED_FACE('',(#974),#522,.F.) ;
#3483=ADVANCED_FACE('',(#975),#523,.T.) ;
#3484=ADVANCED_FACE('',(#976),#524,.F.) ;
#3485=ADVANCED_FACE('',(#977),#525,.T.) ;
#3486=ADVANCED_FACE('',(#978),#526,.F.) ;
#3487=ADVANCED_FACE('',(#979),#158,.T.) ;
#3488=ADVANCED_FACE('',(#980),#159,.F.) ;
#3489=ADVANCED_FACE('',(#981),#527,.F.) ;
#3490=ADVANCED_FACE('',(#982),#528,.F.) ;
#3491=ADVANCED_FACE('',(#983),#529,.F.) ;
#3492=ADVANCED_FACE('',(#984),#530,.T.) ;
#3493=ADVANCED_FACE('',(#985),#531,.F.) ;
#3585=CLOSED_SHELL('',(#3451,#3452,#3453,#3454,#3455,#3456,#3457,#3458,
#3459,#3460,#3461,#3462,#3463,#3464,#3465,#3466,#3467,#3468,#3469,#3470,
#3471,#3472,#3473,#3474,#3475,#3476,#3477,#3478,#3479,#3480,#3481,#3482,
#3483,#3484,#3485,#3486,#3487,#3488,#3489,#3490,#3491,#3492,#3493)) ;
#4170=AXIS2_PLACEMENT_3D('',#9728,#4951,#4952) ;
#4171=AXIS2_PLACEMENT_3D('',#9729,#4953,#4954) ;
#4172=AXIS2_PLACEMENT_3D('',#9731,#4955,#4956) ;
#4173=AXIS2_PLACEMENT_3D('',#9734,#4958,#4959) ;
#4174=AXIS2_PLACEMENT_3D('',#9735,#4960,#4961) ;
#4175=AXIS2_PLACEMENT_3D('',#9752,#4970,#4971) ;
#4176=AXIS2_PLACEMENT_3D('',#9769,#4980,#4981) ;
#4177=AXIS2_PLACEMENT_3D('',#9772,#4984,#4985) ;
#4178=AXIS2_PLACEMENT_3D('',#9775,#4988,#4989) ;
#4179=AXIS2_PLACEMENT_3D('',#9778,#4992,#4993) ;
#4180=AXIS2_PLACEMENT_3D('',#9781,#4996,#4997) ;
#4181=AXIS2_PLACEMENT_3D('',#9785,#4999,#5000) ;
#4182=AXIS2_PLACEMENT_3D('',#9786,#5001,#5002) ;
#4183=AXIS2_PLACEMENT_3D('',#9787,#5003,#5004) ;
#4184=AXIS2_PLACEMENT_3D('',#9789,#5005,#5006) ;
#4185=AXIS2_PLACEMENT_3D('',#9792,#5008,#5009) ;
#4186=AXIS2_PLACEMENT_3D('',#9793,#5010,#5011) ;
#4187=AXIS2_PLACEMENT_3D('',#9795,#5013,#5014) ;
#4188=AXIS2_PLACEMENT_3D('',#9797,#5016,#5017) ;
#4189=AXIS2_PLACEMENT_3D('',#9803,#5021,#5022) ;
#4190=AXIS2_PLACEMENT_3D('',#9809,#5026,#5027) ;
#4191=AXIS2_PLACEMENT_3D('',#9811,#5029,#5030) ;
#4192=AXIS2_PLACEMENT_3D('',#9813,#5032,#5033) ;
#4193=AXIS2_PLACEMENT_3D('',#9814,#5034,#5035) ;
#4194=AXIS2_PLACEMENT_3D('',#9818,#5037,#5038) ;
#4195=AXIS2_PLACEMENT_3D('',#9819,#5039,#5040) ;
#4196=AXIS2_PLACEMENT_3D('',#9820,#5041,#5042) ;
#4197=AXIS2_PLACEMENT_3D('',#9822,#5043,#5044) ;
#4198=AXIS2_PLACEMENT_3D('',#9825,#5046,#5047) ;
#4199=AXIS2_PLACEMENT_3D('',#9826,#5048,#5049) ;
#4200=AXIS2_PLACEMENT_3D('',#9828,#5051,#5052) ;
#4201=AXIS2_PLACEMENT_3D('',#9830,#5054,#5055) ;
#4202=AXIS2_PLACEMENT_3D('',#9836,#5059,#5060) ;
#4203=AXIS2_PLACEMENT_3D('',#9842,#5064,#5065) ;
#4204=AXIS2_PLACEMENT_3D('',#9844,#5067,#5068) ;
#4205=AXIS2_PLACEMENT_3D('',#9846,#5070,#5071) ;
#4206=AXIS2_PLACEMENT_3D('',#9847,#5072,#5073) ;
#4207=AXIS2_PLACEMENT_3D('',#9851,#5075,#5076) ;
#4208=AXIS2_PLACEMENT_3D('',#9852,#5077,#5078) ;
#4209=AXIS2_PLACEMENT_3D('',#9853,#5079,#5080) ;
#4210=AXIS2_PLACEMENT_3D('',#9855,#5081,#5082) ;
#4211=AXIS2_PLACEMENT_3D('',#9858,#5084,#5085) ;
#4212=AXIS2_PLACEMENT_3D('',#9859,#5086,#5087) ;
#4213=AXIS2_PLACEMENT_3D('',#9861,#5089,#5090) ;
#4214=AXIS2_PLACEMENT_3D('',#9863,#5092,#5093) ;
#4215=AXIS2_PLACEMENT_3D('',#9869,#5097,#5098) ;
#4216=AXIS2_PLACEMENT_3D('',#9875,#5102,#5103) ;
#4217=AXIS2_PLACEMENT_3D('',#9877,#5105,#5106) ;
#4218=AXIS2_PLACEMENT_3D('',#9879,#5108,#5109) ;
#4219=AXIS2_PLACEMENT_3D('',#9880,#5110,#5111) ;
#4220=AXIS2_PLACEMENT_3D('',#9884,#5113,#5114) ;
#4221=AXIS2_PLACEMENT_3D('',#9885,#5115,#5116) ;
#4222=AXIS2_PLACEMENT_3D('',#9886,#5117,#5118) ;
#4223=AXIS2_PLACEMENT_3D('',#9888,#5119,#5120) ;
#4224=AXIS2_PLACEMENT_3D('',#9891,#5122,#5123) ;
#4225=AXIS2_PLACEMENT_3D('',#9892,#5124,#5125) ;
#4226=AXIS2_PLACEMENT_3D('',#9894,#5127,#5128) ;
#4227=AXIS2_PLACEMENT_3D('',#9896,#5130,#5131) ;
#4228=AXIS2_PLACEMENT_3D('',#9902,#5135,#5136) ;
#4229=AXIS2_PLACEMENT_3D('',#9908,#5140,#5141) ;
#4230=AXIS2_PLACEMENT_3D('',#9910,#5143,#5144) ;
#4231=AXIS2_PLACEMENT_3D('',#9912,#5146,#5147) ;
#4951=DIRECTION('axis',(0.,0.,1.)) ;
#4952=DIRECTION('refdir',(1.,0.,0.)) ;
#4953=DIRECTION('center_axis',(0.,-1.,-3.49148133884313E-15)) ;
#4954=DIRECTION('ref_axis',(1.,0.,0.)) ;
#4955=DIRECTION('center_axis',(0.,-1.,-3.49148133884313E-15)) ;
#4956=DIRECTION('ref_axis',(1.,0.,0.)) ;
#4957=DIRECTION('',(0.,-1.,-3.49148133884313E-15)) ;
#4958=DIRECTION('center_axis',(0.,-1.,-3.49148133884313E-15)) ;
#4959=DIRECTION('ref_axis',(1.,0.,0.)) ;
#4960=DIRECTION('center_axis',(0.,-1.,-3.49148133884313E-15)) ;
#4961=DIRECTION('ref_axis',(1.,0.,0.)) ;
#4962=DIRECTION('',(0.,-3.49148133884313E-15,1.)) ;
#4963=DIRECTION('',(-0.707106781186548,2.46885013108227E-15,-0.707106781186548)) ;
#4964=DIRECTION('',(1.,-4.62017040814388E-31,1.32326939764619E-16)) ;
#4965=DIRECTION('',(-0.707106781186548,-2.46885013108227E-15,0.707106781186548)) ;
#4966=DIRECTION('',(0.,3.49148133884313E-15,-1.)) ;
#4967=DIRECTION('',(0.707106781186547,-2.46885013108227E-15,0.707106781186547)) ;
#4968=DIRECTION('',(-1.,4.62017040814388E-31,-1.32326939764619E-16)) ;
#4969=DIRECTION('',(0.707106781186549,2.46885013108226E-15,-0.707106781186546)) ;
#4970=DIRECTION('center_axis',(0.,-1.,-3.49148133884313E-15)) ;
#4971=DIRECTION('ref_axis',(1.,0.,0.)) ;
#4972=DIRECTION('',(1.,-4.62017040814388E-31,1.32326939764619E-16)) ;
#4973=DIRECTION('',(0.707106781186548,-2.46885013108227E-15,0.707106781186548)) ;
#4974=DIRECTION('',(0.,-3.49148133884313E-15,1.)) ;
#4975=DIRECTION('',(-0.707106781186549,-2.46885013108226E-15,0.707106781186546)) ;
#4976=DIRECTION('',(-1.,4.62017040814388E-31,-1.32326939764619E-16)) ;
#4977=DIRECTION('',(-0.707106781186548,2.46885013108227E-15,-0.707106781186548)) ;
#4978=DIRECTION('',(0.,3.49148133884313E-15,-1.)) ;
#4979=DIRECTION('',(0.707106781186547,2.46885013108227E-15,-0.707106781186547)) ;
#4980=DIRECTION('center_axis',(-0.707106781186548,-2.46885013108227E-15,
0.707106781186548)) ;
#4981=DIRECTION('ref_axis',(3.82771347986811E-30,-1.,-3.49148133884313E-15)) ;
#4982=DIRECTION('',(0.,1.,3.49148133884313E-15)) ;
#4983=DIRECTION('',(0.,-1.,-3.49148133884313E-15)) ;
#4984=DIRECTION('center_axis',(0.707106781186548,-2.46885013108227E-15,
0.707106781186548)) ;
#4985=DIRECTION('ref_axis',(-3.82771347986811E-30,-1.,-3.49148133884313E-15)) ;
#4986=DIRECTION('',(0.,1.,3.49148133884313E-15)) ;
#4987=DIRECTION('',(0.,-1.,-3.49148133884313E-15)) ;
#4988=DIRECTION('center_axis',(0.707106781186548,2.46885013108227E-15,-0.707106781186548)) ;
#4989=DIRECTION('ref_axis',(3.82771347986811E-30,-1.,-3.49148133884313E-15)) ;
#4990=DIRECTION('',(0.,1.,3.49148133884313E-15)) ;
#4991=DIRECTION('',(0.,-1.,-3.49148133884313E-15)) ;
#4992=DIRECTION('center_axis',(-0.707106781186546,2.46885013108227E-15,
-0.707106781186549)) ;
#4993=DIRECTION('ref_axis',(-1.32640682077634E-30,-1.,-3.49148133884313E-15)) ;
#4994=DIRECTION('',(0.,1.,3.49148133884313E-15)) ;
#4995=DIRECTION('',(0.,-1.,-3.49148133884313E-15)) ;
#4996=DIRECTION('center_axis',(-1.,0.,0.)) ;
#4997=DIRECTION('ref_axis',(0.,-1.,-3.49148133884313E-15)) ;
#4998=DIRECTION('',(-1.38951567537567E-16,-5.77315972805081E-15,1.)) ;
#4999=DIRECTION('center_axis',(-1.,0.,0.)) ;
#5000=DIRECTION('ref_axis',(0.,1.,0.)) ;
#5001=DIRECTION('center_axis',(-1.,0.,0.)) ;
#5002=DIRECTION('ref_axis',(0.,1.,0.)) ;
#5003=DIRECTION('center_axis',(-1.,0.,0.)) ;
#5004=DIRECTION('ref_axis',(0.,-1.,-3.49148133884313E-15)) ;
#5005=DIRECTION('center_axis',(1.,0.,0.)) ;
#5006=DIRECTION('ref_axis',(0.,1.,0.)) ;
#5007=DIRECTION('',(-1.38951567537567E-16,-5.77315972805081E-15,1.)) ;
#5008=DIRECTION('center_axis',(1.,0.,0.)) ;
#5009=DIRECTION('ref_axis',(0.,1.,0.)) ;
#5010=DIRECTION('center_axis',(1.,0.,0.)) ;
#5011=DIRECTION('ref_axis',(0.,-1.00929365875017E-14,1.)) ;
#5012=DIRECTION('',(-1.,4.85146805060415E-31,-1.38951567537567E-16)) ;
#5013=DIRECTION('center_axis',(1.,0.,0.)) ;
#5014=DIRECTION('ref_axis',(0.,0.,1.)) ;
#5015=DIRECTION('',(1.,-4.85146805060415E-31,1.38951567537567E-16)) ;
#5016=DIRECTION('center_axis',(-1.,8.13374953119913E-31,-1.38951567537567E-16)) ;
#5017=DIRECTION('ref_axis',(1.38951567537567E-16,3.49148133884313E-15,-1.)) ;
#5018=DIRECTION('',(4.37905770101505E-47,1.,5.85365798698176E-15)) ;
#5019=DIRECTION('',(1.38951567537567E-16,6.98296267768627E-15,-1.)) ;
#5020=DIRECTION('',(4.37905770101505E-47,1.,5.85365798698176E-15)) ;
#5021=DIRECTION('center_axis',(1.,-8.13374953119913E-31,1.38951567537567E-16)) ;
#5022=DIRECTION('ref_axis',(-1.38951567537567E-16,-3.49148133884313E-15,
1.)) ;
#5023=DIRECTION('',(-4.37905770101505E-47,-1.,-5.85365798698176E-15)) ;
#5024=DIRECTION('',(1.38951567537567E-16,6.98296267768627E-15,-1.)) ;
#5025=DIRECTION('',(-4.37905770101505E-47,-1.,-5.85365798698176E-15)) ;
#5026=DIRECTION('center_axis',(1.38951567537567E-16,5.85365798698176E-15,
-1.)) ;
#5027=DIRECTION('ref_axis',(0.,1.,5.85365798698176E-15)) ;
#5028=DIRECTION('',(-1.,4.85146805060415E-31,-1.38951567537567E-16)) ;
#5029=DIRECTION('center_axis',(1.38951567537567E-16,5.85365798698176E-15,
-1.)) ;
#5030=DIRECTION('ref_axis',(0.,1.,5.85365798698176E-15)) ;
#5031=DIRECTION('',(-1.,4.85146805060415E-31,-1.38951567537567E-16)) ;
#5032=DIRECTION('center_axis',(4.85146805060415E-31,-1.,-6.98296267768627E-15)) ;
#5033=DIRECTION('ref_axis',(1.36633227546431E-61,6.98296267768627E-15,-1.)) ;
#5034=DIRECTION('center_axis',(0.,-3.38306112159458E-15,1.)) ;
#5035=DIRECTION('ref_axis',(0.,-1.,-3.38306112159458E-15)) ;
#5036=DIRECTION('',(1.,-2.28167838920768E-15,-7.96643751716028E-30)) ;
#5037=DIRECTION('center_axis',(0.,-3.38306112159458E-15,1.)) ;
#5038=DIRECTION('ref_axis',(0.,1.,3.38306112159458E-15)) ;
#5039=DIRECTION('center_axis',(0.,-3.38306112159458E-15,1.)) ;
#5040=DIRECTION('ref_axis',(0.,1.,3.38306112159458E-15)) ;
#5041=DIRECTION('center_axis',(0.,-3.38306112159458E-15,1.)) ;
#5042=DIRECTION('ref_axis',(0.,-1.,-3.38306112159458E-15)) ;
#5043=DIRECTION('center_axis',(0.,3.38306112159458E-15,-1.)) ;
#5044=DIRECTION('ref_axis',(0.,1.,3.38306112159458E-15)) ;
#5045=DIRECTION('',(1.,-2.28167838920768E-15,-7.96643751716028E-30)) ;
#5046=DIRECTION('center_axis',(0.,3.38306112159458E-15,-1.)) ;
#5047=DIRECTION('ref_axis',(0.,1.,3.38306112159458E-15)) ;
#5048=DIRECTION('center_axis',(0.,3.38306112159458E-15,-1.)) ;
#5049=DIRECTION('ref_axis',(1.,0.,0.)) ;
#5050=DIRECTION('',(1.64114074029749E-31,-3.42200555507435E-15,1.)) ;
#5051=DIRECTION('center_axis',(0.,3.38306112159458E-15,-1.)) ;
#5052=DIRECTION('ref_axis',(1.,0.,0.)) ;
#5053=DIRECTION('',(-1.64114074029749E-31,3.42200555507435E-15,-1.)) ;
#5054=DIRECTION('center_axis',(0.,-3.49148133884313E-15,1.)) ;
#5055=DIRECTION('ref_axis',(0.,-1.,-3.49148133884313E-15)) ;
#5056=DIRECTION('',(2.36217664813863E-15,1.,3.49148133884313E-15)) ;
#5057=DIRECTION('',(-1.,3.49148133884313E-15,1.21904419394898E-29)) ;
#5058=DIRECTION('',(2.36217664813863E-15,1.,3.49148133884313E-15)) ;
#5059=DIRECTION('center_axis',(0.,3.49148133884313E-15,-1.)) ;
#5060=DIRECTION('ref_axis',(0.,1.,3.49148133884313E-15)) ;
#5061=DIRECTION('',(-2.36217664813863E-15,-1.,-3.49148133884313E-15)) ;
#5062=DIRECTION('',(-1.,3.49148133884313E-15,1.21904419394898E-29)) ;
#5063=DIRECTION('',(-2.36217664813863E-15,-1.,-3.49148133884313E-15)) ;
#5064=DIRECTION('center_axis',(-1.,2.36217664813863E-15,8.24749568602705E-30)) ;
#5065=DIRECTION('ref_axis',(-2.36217664813863E-15,-1.,-3.49148133884313E-15)) ;
#5066=DIRECTION('',(0.,-3.49148133884313E-15,1.)) ;
#5067=DIRECTION('center_axis',(-1.,2.36217664813863E-15,8.24749568602705E-30)) ;
#5068=DIRECTION('ref_axis',(-2.36217664813863E-15,-1.,-3.49148133884313E-15)) ;
#5069=DIRECTION('',(0.,-3.49148133884313E-15,1.)) ;
#5070=DIRECTION('center_axis',(-3.49148133884313E-15,-1.,-3.49148133884313E-15)) ;
#5071=DIRECTION('ref_axis',(1.,-3.49148133884313E-15,-1.21904419394898E-29)) ;
#5072=DIRECTION('center_axis',(1.,0.,0.)) ;
#5073=DIRECTION('ref_axis',(0.,1.,3.49148133884313E-15)) ;
#5074=DIRECTION('',(1.38951567537567E-16,1.20980294963545E-15,-1.)) ;
#5075=DIRECTION('center_axis',(1.,0.,0.)) ;
#5076=DIRECTION('ref_axis',(0.,-1.,-1.38777878078146E-14)) ;
#5077=DIRECTION('center_axis',(1.,0.,0.)) ;
#5078=DIRECTION('ref_axis',(0.,-1.,-1.00929365875015E-14)) ;
#5079=DIRECTION('center_axis',(1.,0.,0.)) ;
#5080=DIRECTION('ref_axis',(0.,1.,3.49148133884313E-15)) ;
#5081=DIRECTION('center_axis',(-1.,0.,0.)) ;
#5082=DIRECTION('ref_axis',(0.,-1.,0.)) ;
#5083=DIRECTION('',(1.38951567537567E-16,1.20980294963545E-15,-1.)) ;
#5084=DIRECTION('center_axis',(-1.,0.,0.)) ;
#5085=DIRECTION('ref_axis',(0.,-1.,0.)) ;
#5086=DIRECTION('center_axis',(-1.,0.,0.)) ;
#5087=DIRECTION('ref_axis',(0.,0.,-1.)) ;
#5088=DIRECTION('',(1.,-4.85146805060415E-31,1.38951567537567E-16)) ;
#5089=DIRECTION('center_axis',(-1.,0.,0.)) ;
#5090=DIRECTION('ref_axis',(0.,0.,-1.)) ;
#5091=DIRECTION('',(-1.,4.85146805060415E-31,-1.38951567537567E-16)) ;
#5092=DIRECTION('center_axis',(1.,-1.56918657000917E-31,1.38951567537567E-16)) ;
#5093=DIRECTION('ref_axis',(-1.38951567537567E-16,-3.49148133884313E-15,
1.)) ;
#5094=DIRECTION('',(0.,1.,1.1293046907045E-15)) ;
#5095=DIRECTION('',(-1.38951567537567E-16,0.,1.)) ;
#5096=DIRECTION('',(0.,1.,1.1293046907045E-15)) ;
#5097=DIRECTION('center_axis',(-1.,1.56918657000917E-31,-1.38951567537567E-16)) ;
#5098=DIRECTION('ref_axis',(1.38951567537567E-16,3.49148133884313E-15,-1.)) ;
#5099=DIRECTION('',(0.,-1.,-1.1293046907045E-15)) ;
#5100=DIRECTION('',(-1.38951567537567E-16,0.,1.)) ;
#5101=DIRECTION('',(0.,-1.,-1.1293046907045E-15)) ;
#5102=DIRECTION('center_axis',(-1.38951567537567E-16,-1.1293046907045E-15,
1.)) ;
#5103=DIRECTION('ref_axis',(0.,-1.,-1.1293046907045E-15)) ;
#5104=DIRECTION('',(1.,-4.85146805060415E-31,1.38951567537567E-16)) ;
#5105=DIRECTION('center_axis',(-1.38951567537567E-16,-1.1293046907045E-15,
1.)) ;
#5106=DIRECTION('ref_axis',(0.,-1.,-1.1293046907045E-15)) ;
#5107=DIRECTION('',(1.,-4.85146805060415E-31,1.38951567537567E-16)) ;
#5108=DIRECTION('center_axis',(-4.85146805060415E-31,-1.,0.)) ;
#5109=DIRECTION('ref_axis',(0.,0.,-1.)) ;
#5110=DIRECTION('center_axis',(0.,3.49148133884313E-15,-1.)) ;
#5111=DIRECTION('ref_axis',(0.,1.,3.49148133884313E-15)) ;
#5112=DIRECTION('',(-1.,-2.28167838920768E-15,-7.96643751716028E-30)) ;
#5113=DIRECTION('center_axis',(0.,3.49148133884313E-15,-1.)) ;
#5114=DIRECTION('ref_axis',(0.,-1.,-3.49148133884313E-15)) ;
#5115=DIRECTION('center_axis',(0.,3.49148133884313E-15,-1.)) ;
#5116=DIRECTION('ref_axis',(0.,-1.,-3.49148133884313E-15)) ;
#5117=DIRECTION('center_axis',(0.,3.49148133884313E-15,-1.)) ;
#5118=DIRECTION('ref_axis',(0.,1.,3.49148133884313E-15)) ;
#5119=DIRECTION('center_axis',(0.,-3.49148133884313E-15,1.)) ;
#5120=DIRECTION('ref_axis',(0.,-1.,-3.49148133884313E-15)) ;
#5121=DIRECTION('',(-1.,-2.28167838920768E-15,-7.96643751716028E-30)) ;
#5122=DIRECTION('center_axis',(0.,-3.49148133884313E-15,1.)) ;
#5123=DIRECTION('ref_axis',(0.,-1.,-3.49148133884313E-15)) ;
#5124=DIRECTION('center_axis',(0.,-3.49148133884313E-15,1.)) ;
#5125=DIRECTION('ref_axis',(-1.,0.,0.)) ;
#5126=DIRECTION('',(0.,3.49148133884313E-15,-1.)) ;
#5127=DIRECTION('center_axis',(0.,-3.49148133884313E-15,1.)) ;
#5128=DIRECTION('ref_axis',(-1.,0.,0.)) ;
#5129=DIRECTION('',(0.,-3.49148133884313E-15,1.)) ;
#5130=DIRECTION('center_axis',(0.,3.49148133884313E-15,-1.)) ;
#5131=DIRECTION('ref_axis',(0.,1.,3.49148133884313E-15)) ;
#5132=DIRECTION('',(-2.36217664813863E-15,1.,3.49148133884313E-15)) ;
#5133=DIRECTION('',(1.,3.49148133884313E-15,1.21904419394898E-29)) ;
#5134=DIRECTION('',(-2.36217664813863E-15,1.,3.49148133884313E-15)) ;
#5135=DIRECTION('center_axis',(0.,-3.49148133884313E-15,1.)) ;
#5136=DIRECTION('ref_axis',(0.,-1.,-3.49148133884313E-15)) ;
#5137=DIRECTION('',(2.36217664813863E-15,-1.,-3.49148133884313E-15)) ;
#5138=DIRECTION('',(1.,3.49148133884313E-15,1.21904419394898E-29)) ;
#5139=DIRECTION('',(2.36217664813863E-15,-1.,-3.49148133884313E-15)) ;
#5140=DIRECTION('center_axis',(1.,2.36217664813863E-15,8.24749568602705E-30)) ;
#5141=DIRECTION('ref_axis',(-2.36217664813863E-15,1.,3.49148133884313E-15)) ;
#5142=DIRECTION('',(0.,3.49148133884313E-15,-1.)) ;
#5143=DIRECTION('center_axis',(1.,2.36217664813863E-15,8.24749568602705E-30)) ;
#5144=DIRECTION('ref_axis',(-2.36217664813863E-15,1.,3.49148133884313E-15)) ;
#5145=DIRECTION('',(0.,3.49148133884313E-15,-1.)) ;
#5146=DIRECTION('center_axis',(3.49148133884313E-15,-1.,-3.49148133884313E-15)) ;
#5147=DIRECTION('ref_axis',(1.,3.49148133884313E-15,1.21904419394898E-29)) ;
#9728=CARTESIAN_POINT('',(0.,0.,0.)) ;
#9729=CARTESIAN_POINT('Origin',(23.47768801576,41.8330586252738,68.2224337399912)) ;
#9730=CARTESIAN_POINT('',(-17.5327992399109,40.9830586252738,68.2224337399912)) ;
#9731=CARTESIAN_POINT('Origin',(23.47768801576,40.9830586252738,68.2224337399912)) ;
#9732=CARTESIAN_POINT('',(-17.5327992399109,40.8330586252738,68.2224337399912)) ;
#9733=CARTESIAN_POINT('',(-17.5327992399108,41.8330586252738,68.2224337399912)) ;
#9734=CARTESIAN_POINT('Origin',(23.47768801576,40.8330586252738,68.2224337399912)) ;
#9735=CARTESIAN_POINT('Origin',(23.47768801576,40.9830586252738,68.222433740001)) ;
#9736=CARTESIAN_POINT('',(65.42768801576,40.983058625274,28.272433740001)) ;
#9737=CARTESIAN_POINT('',(65.42768801576,40.9830586252737,108.172433740001)) ;
#9738=CARTESIAN_POINT('',(65.42768801576,40.983058625274,26.272433740001)) ;
#9739=CARTESIAN_POINT('',(63.42768801576,40.983058625274,26.272433740001)) ;
#9740=CARTESIAN_POINT('',(63.42768801576,40.983058625274,26.272433740001)) ;
#9741=CARTESIAN_POINT('',(-16.47231198424,40.983058625274,26.272433740001)) ;
#9742=CARTESIAN_POINT('',(65.42768801576,40.983058625274,26.272433740001)) ;
#9743=CARTESIAN_POINT('',(-18.47231198424,40.983058625274,28.272433740001)) ;
#9744=CARTESIAN_POINT('',(-18.47231198424,40.983058625274,28.272433740001)) ;
#9745=CARTESIAN_POINT('',(-18.47231198424,40.9830586252737,108.172433740001)) ;
#9746=CARTESIAN_POINT('',(-18.47231198424,40.983058625274,26.272433740001)) ;
#9747=CARTESIAN_POINT('',(-16.47231198424,40.9830586252737,110.172433740001)) ;
#9748=CARTESIAN_POINT('',(-16.47231198424,40.9830586252737,110.172433740001)) ;
#9749=CARTESIAN_POINT('',(63.4276880157599,40.9830586252737,110.172433740001)) ;
#9750=CARTESIAN_POINT('',(65.42768801576,40.9830586252737,110.172433740001)) ;
#9751=CARTESIAN_POINT('',(65.42768801576,40.9830586252737,108.172433740001)) ;
#9752=CARTESIAN_POINT('Origin',(23.47768801576,40.8330586252738,68.222433740001)) ;
#9753=CARTESIAN_POINT('',(-16.47231198424,40.833058625274,26.272433740001)) ;
#9754=CARTESIAN_POINT('',(63.42768801576,40.833058625274,26.272433740001)) ;
#9755=CARTESIAN_POINT('',(65.42768801576,40.833058625274,26.272433740001)) ;
#9756=CARTESIAN_POINT('',(65.42768801576,40.833058625274,28.272433740001)) ;
#9757=CARTESIAN_POINT('',(64.4276880157599,40.833058625274,27.272433740001)) ;
#9758=CARTESIAN_POINT('',(65.42768801576,40.8330586252737,108.172433740001)) ;
#9759=CARTESIAN_POINT('',(65.42768801576,40.833058625274,26.272433740001)) ;
#9760=CARTESIAN_POINT('',(63.4276880157599,40.8330586252737,110.172433740001)) ;
#9761=CARTESIAN_POINT('',(64.4276880157598,40.8330586252737,109.172433740001)) ;
#9762=CARTESIAN_POINT('',(-16.47231198424,40.8330586252737,110.172433740001)) ;
#9763=CARTESIAN_POINT('',(65.42768801576,40.8330586252737,110.172433740001)) ;
#9764=CARTESIAN_POINT('',(-18.47231198424,40.8330586252737,108.172433740001)) ;
#9765=CARTESIAN_POINT('',(-17.47231198424,40.8330586252737,109.172433740001)) ;
#9766=CARTESIAN_POINT('',(-18.47231198424,40.833058625274,28.272433740001)) ;
#9767=CARTESIAN_POINT('',(-18.47231198424,40.833058625274,26.272433740001)) ;
#9768=CARTESIAN_POINT('',(-17.47231198424,40.833058625274,27.272433740001)) ;
#9769=CARTESIAN_POINT('Origin',(63.42768801576,40.983058625274,26.272433740001)) ;
#9770=CARTESIAN_POINT('',(65.42768801576,40.983058625274,28.272433740001)) ;
#9771=CARTESIAN_POINT('',(63.42768801576,40.983058625274,26.272433740001)) ;
#9772=CARTESIAN_POINT('Origin',(-18.47231198424,40.983058625274,28.272433740001)) ;
#9773=CARTESIAN_POINT('',(-16.47231198424,40.983058625274,26.272433740001)) ;
#9774=CARTESIAN_POINT('',(-18.47231198424,40.983058625274,28.272433740001)) ;
#9775=CARTESIAN_POINT('Origin',(-16.47231198424,40.9830586252737,110.172433740001)) ;
#9776=CARTESIAN_POINT('',(-18.47231198424,40.9830586252737,108.172433740001)) ;
#9777=CARTESIAN_POINT('',(-16.47231198424,40.9830586252737,110.172433740001)) ;
#9778=CARTESIAN_POINT('Origin',(65.42768801576,40.9830586252737,108.172433740001)) ;
#9779=CARTESIAN_POINT('',(63.4276880157599,40.9830586252737,110.172433740001)) ;
#9780=CARTESIAN_POINT('',(65.42768801576,40.9830586252737,108.172433740001)) ;
#9781=CARTESIAN_POINT('Origin',(-16.47231198424,41.3830586252737,110.172433740001)) ;
#9782=CARTESIAN_POINT('',(-16.47231198424,41.3830586252737,110.572433740001)) ;
#9783=CARTESIAN_POINT('',(-16.47231198424,41.3830586252737,110.722433740001)) ;
#9784=CARTESIAN_POINT('',(-16.47231198424,41.3830586252737,110.722433740001)) ;
#9785=CARTESIAN_POINT('Origin',(-16.47231198424,41.3830586252737,110.172433740001)) ;
#9786=CARTESIAN_POINT('Origin',(-16.47231198424,41.3830586252737,110.172433740001)) ;
#9787=CARTESIAN_POINT('Origin',(63.4276880157599,41.3830586252737,110.172433740001)) ;
#9788=CARTESIAN_POINT('',(63.4276880157599,41.3830586252737,110.572433740001)) ;
#9789=CARTESIAN_POINT('Origin',(63.4276880157599,41.3830586252737,110.172433740001)) ;
#9790=CARTESIAN_POINT('',(63.4276880157599,41.3830586252737,110.722433740001)) ;
#9791=CARTESIAN_POINT('',(63.4276880157599,41.3830586252737,110.572433740001)) ;
#9792=CARTESIAN_POINT('Origin',(63.4276880157599,41.3830586252737,110.172433740001)) ;
#9793=CARTESIAN_POINT('Origin',(63.4276880157599,41.3830586252737,110.172433740001)) ;
#9794=CARTESIAN_POINT('',(-16.47231198424,41.3830586252737,110.722433740001)) ;
#9795=CARTESIAN_POINT('Origin',(63.4276880157599,41.3830586252737,110.172433740001)) ;
#9796=CARTESIAN_POINT('',(-16.47231198424,41.3830586252737,110.572433740001)) ;
#9797=CARTESIAN_POINT('Origin',(63.4276880157599,43.3330586252737,110.722433740001)) ;
#9798=CARTESIAN_POINT('',(63.4276880157599,43.3330586252737,110.572433740001)) ;
#9799=CARTESIAN_POINT('',(63.4276880157599,43.3330586252737,110.572433740001)) ;
#9800=CARTESIAN_POINT('',(63.4276880157599,43.3330586252737,110.722433740001)) ;
#9801=CARTESIAN_POINT('',(63.4276880157599,43.3330586252737,110.722433740001)) ;
#9802=CARTESIAN_POINT('',(63.4276880157599,40.8330586252736,110.722433740001)) ;
#9803=CARTESIAN_POINT('Origin',(-16.47231198424,40.9830586252737,110.722433740001)) ;
#9804=CARTESIAN_POINT('',(-16.47231198424,43.3330586252737,110.722433740001)) ;
#9805=CARTESIAN_POINT('',(-16.47231198424,40.8330586252736,110.722433740001)) ;
#9806=CARTESIAN_POINT('',(-16.47231198424,43.3330586252737,110.572433740001)) ;
#9807=CARTESIAN_POINT('',(-16.47231198424,43.3330586252737,110.722433740001)) ;
#9808=CARTESIAN_POINT('',(-16.47231198424,40.9830586252737,110.572433740001)) ;
#9809=CARTESIAN_POINT('Origin',(23.4776880157599,40.8330586252736,110.722433740001)) ;
#9810=CARTESIAN_POINT('',(23.4776880157599,43.3330586252737,110.722433740001)) ;
#9811=CARTESIAN_POINT('Origin',(23.4776880157599,40.8330586252736,110.572433740001)) ;
#9812=CARTESIAN_POINT('',(-16.47231198424,43.3330586252737,110.572433740001)) ;
#9813=CARTESIAN_POINT('Origin',(-16.47231198424,43.3330586252737,110.722433740001)) ;
#9814=CARTESIAN_POINT('Origin',(65.42768801576,41.3830586252737,108.172433740001)) ;
#9815=CARTESIAN_POINT('',(65.82768801576,41.3830586252737,108.172433740001)) ;
#9816=CARTESIAN_POINT('',(65.97768801576,41.3830586252737,108.172433740001)) ;
#9817=CARTESIAN_POINT('',(65.97768801576,41.3830586252737,108.172433740001)) ;
#9818=CARTESIAN_POINT('Origin',(65.42768801576,41.3830586252737,108.172433740001)) ;
#9819=CARTESIAN_POINT('Origin',(65.42768801576,41.3830586252737,108.172433740001)) ;
#9820=CARTESIAN_POINT('Origin',(65.42768801576,41.383058625274,28.272433740001)) ;
#9821=CARTESIAN_POINT('',(65.82768801576,41.383058625274,28.272433740001)) ;
#9822=CARTESIAN_POINT('Origin',(65.42768801576,41.383058625274,28.272433740001)) ;
#9823=CARTESIAN_POINT('',(65.97768801576,41.383058625274,28.272433740001)) ;
#9824=CARTESIAN_POINT('',(65.82768801576,41.383058625274,28.272433740001)) ;
#9825=CARTESIAN_POINT('Origin',(65.42768801576,41.383058625274,28.272433740001)) ;
#9826=CARTESIAN_POINT('Origin',(65.42768801576,41.383058625274,28.272433740001)) ;
#9827=CARTESIAN_POINT('',(65.97768801576,41.3830586252737,108.172433740001)) ;
#9828=CARTESIAN_POINT('Origin',(65.42768801576,41.383058625274,28.272433740001)) ;
#9829=CARTESIAN_POINT('',(65.82768801576,41.3830586252737,108.172433740001)) ;
#9830=CARTESIAN_POINT('Origin',(65.97768801576,43.333058625274,28.272433740001)) ;
#9831=CARTESIAN_POINT('',(65.82768801576,43.333058625274,28.272433740001)) ;
#9832=CARTESIAN_POINT('',(65.82768801576,43.333058625274,28.272433740001)) ;
#9833=CARTESIAN_POINT('',(65.97768801576,43.333058625274,28.272433740001)) ;
#9834=CARTESIAN_POINT('',(65.97768801576,43.333058625274,28.272433740001)) ;
#9835=CARTESIAN_POINT('',(65.97768801576,40.8330586252739,28.272433740001)) ;
#9836=CARTESIAN_POINT('Origin',(65.97768801576,40.9830586252737,108.172433740001)) ;
#9837=CARTESIAN_POINT('',(65.97768801576,43.3330586252737,108.172433740001)) ;
#9838=CARTESIAN_POINT('',(65.97768801576,40.8330586252736,108.172433740001)) ;
#9839=CARTESIAN_POINT('',(65.82768801576,43.3330586252737,108.172433740001)) ;
#9840=CARTESIAN_POINT('',(65.97768801576,43.3330586252737,108.172433740001)) ;
#9841=CARTESIAN_POINT('',(65.82768801576,40.9830586252737,108.172433740001)) ;
#9842=CARTESIAN_POINT('Origin',(65.97768801576,40.8330586252737,68.222433740001)) ;
#9843=CARTESIAN_POINT('',(65.97768801576,43.3330586252738,68.222433740001)) ;
#9844=CARTESIAN_POINT('Origin',(65.82768801576,40.8330586252737,68.222433740001)) ;
#9845=CARTESIAN_POINT('',(65.82768801576,43.3330586252737,108.172433740001)) ;
#9846=CARTESIAN_POINT('Origin',(65.97768801576,43.3330586252737,108.172433740001)) ;
#9847=CARTESIAN_POINT('Origin',(63.42768801576,41.383058625274,26.272433740001)) ;
#9848=CARTESIAN_POINT('',(63.42768801576,41.383058625274,25.872433740001)) ;
#9849=CARTESIAN_POINT('',(63.42768801576,41.383058625274,25.722433740001)) ;
#9850=CARTESIAN_POINT('',(63.42768801576,41.383058625274,25.722433740001)) ;
#9851=CARTESIAN_POINT('Origin',(63.42768801576,41.383058625274,26.272433740001)) ;
#9852=CARTESIAN_POINT('Origin',(63.42768801576,41.383058625274,26.272433740001)) ;
#9853=CARTESIAN_POINT('Origin',(-16.47231198424,41.383058625274,26.272433740001)) ;
#9854=CARTESIAN_POINT('',(-16.47231198424,41.383058625274,25.872433740001)) ;
#9855=CARTESIAN_POINT('Origin',(-16.47231198424,41.383058625274,26.272433740001)) ;
#9856=CARTESIAN_POINT('',(-16.47231198424,41.383058625274,25.722433740001)) ;
#9857=CARTESIAN_POINT('',(-16.47231198424,41.383058625274,25.872433740001)) ;
#9858=CARTESIAN_POINT('Origin',(-16.47231198424,41.383058625274,26.272433740001)) ;
#9859=CARTESIAN_POINT('Origin',(-16.47231198424,41.383058625274,26.272433740001)) ;
#9860=CARTESIAN_POINT('',(63.42768801576,41.383058625274,25.722433740001)) ;
#9861=CARTESIAN_POINT('Origin',(-16.47231198424,41.383058625274,26.272433740001)) ;
#9862=CARTESIAN_POINT('',(63.42768801576,41.383058625274,25.872433740001)) ;
#9863=CARTESIAN_POINT('Origin',(-16.47231198424,43.333058625274,25.722433740001)) ;
#9864=CARTESIAN_POINT('',(-16.47231198424,43.333058625274,25.872433740001)) ;
#9865=CARTESIAN_POINT('',(-16.47231198424,43.333058625274,25.872433740001)) ;
#9866=CARTESIAN_POINT('',(-16.47231198424,43.333058625274,25.722433740001)) ;
#9867=CARTESIAN_POINT('',(-16.47231198424,43.333058625274,25.722433740001)) ;
#9868=CARTESIAN_POINT('',(-16.47231198424,40.8330586252739,25.722433740001)) ;
#9869=CARTESIAN_POINT('Origin',(63.42768801576,40.983058625274,25.722433740001)) ;
#9870=CARTESIAN_POINT('',(63.42768801576,43.333058625274,25.722433740001)) ;
#9871=CARTESIAN_POINT('',(63.42768801576,40.8330586252739,25.722433740001)) ;
#9872=CARTESIAN_POINT('',(63.42768801576,43.333058625274,25.872433740001)) ;
#9873=CARTESIAN_POINT('',(63.42768801576,43.333058625274,25.722433740001)) ;
#9874=CARTESIAN_POINT('',(63.42768801576,40.983058625274,25.872433740001)) ;
#9875=CARTESIAN_POINT('Origin',(23.47768801576,40.8330586252739,25.722433740001)) ;
#9876=CARTESIAN_POINT('',(23.47768801576,43.333058625274,25.722433740001)) ;
#9877=CARTESIAN_POINT('Origin',(23.47768801576,40.8330586252739,25.872433740001)) ;
#9878=CARTESIAN_POINT('',(63.42768801576,43.333058625274,25.872433740001)) ;
#9879=CARTESIAN_POINT('Origin',(63.42768801576,43.333058625274,25.722433740001)) ;
#9880=CARTESIAN_POINT('Origin',(-18.47231198424,41.383058625274,28.272433740001)) ;
#9881=CARTESIAN_POINT('',(-18.87231198424,41.383058625274,28.272433740001)) ;
#9882=CARTESIAN_POINT('',(-19.02231198424,41.383058625274,28.272433740001)) ;
#9883=CARTESIAN_POINT('',(-19.02231198424,41.383058625274,28.272433740001)) ;
#9884=CARTESIAN_POINT('Origin',(-18.47231198424,41.383058625274,28.272433740001)) ;
#9885=CARTESIAN_POINT('Origin',(-18.47231198424,41.383058625274,28.272433740001)) ;
#9886=CARTESIAN_POINT('Origin',(-18.47231198424,41.3830586252737,108.172433740001)) ;
#9887=CARTESIAN_POINT('',(-18.87231198424,41.3830586252737,108.172433740001)) ;
#9888=CARTESIAN_POINT('Origin',(-18.47231198424,41.3830586252737,108.172433740001)) ;
#9889=CARTESIAN_POINT('',(-19.02231198424,41.3830586252737,108.172433740001)) ;
#9890=CARTESIAN_POINT('',(-18.87231198424,41.3830586252737,108.172433740001)) ;
#9891=CARTESIAN_POINT('Origin',(-18.47231198424,41.3830586252737,108.172433740001)) ;
#9892=CARTESIAN_POINT('Origin',(-18.47231198424,41.3830586252737,108.172433740001)) ;
#9893=CARTESIAN_POINT('',(-19.02231198424,41.383058625274,28.272433740001)) ;
#9894=CARTESIAN_POINT('Origin',(-18.47231198424,41.3830586252737,108.172433740001)) ;
#9895=CARTESIAN_POINT('',(-18.87231198424,41.383058625274,28.272433740001)) ;
#9896=CARTESIAN_POINT('Origin',(-19.02231198424,43.3330586252737,108.172433740001)) ;
#9897=CARTESIAN_POINT('',(-18.87231198424,43.3330586252737,108.172433740001)) ;
#9898=CARTESIAN_POINT('',(-18.87231198424,43.3330586252737,108.172433740001)) ;
#9899=CARTESIAN_POINT('',(-19.02231198424,43.3330586252737,108.172433740001)) ;
#9900=CARTESIAN_POINT('',(-19.02231198424,43.3330586252737,108.172433740001)) ;
#9901=CARTESIAN_POINT('',(-19.02231198424,40.8330586252736,108.172433740001)) ;
#9902=CARTESIAN_POINT('Origin',(-19.02231198424,40.983058625274,28.272433740001)) ;
#9903=CARTESIAN_POINT('',(-19.02231198424,43.333058625274,28.272433740001)) ;
#9904=CARTESIAN_POINT('',(-19.02231198424,40.8330586252739,28.272433740001)) ;
#9905=CARTESIAN_POINT('',(-18.87231198424,43.333058625274,28.272433740001)) ;
#9906=CARTESIAN_POINT('',(-19.02231198424,43.333058625274,28.272433740001)) ;
#9907=CARTESIAN_POINT('',(-18.87231198424,40.983058625274,28.272433740001)) ;
#9908=CARTESIAN_POINT('Origin',(-19.02231198424,40.8330586252737,68.222433740001)) ;
#9909=CARTESIAN_POINT('',(-19.02231198424,43.3330586252738,68.222433740001)) ;
#9910=CARTESIAN_POINT('Origin',(-18.87231198424,40.8330586252737,68.222433740001)) ;
#9911=CARTESIAN_POINT('',(-18.87231198424,43.333058625274,28.272433740001)) ;
#9912=CARTESIAN_POINT('Origin',(-19.02231198424,43.333058625274,28.272433740001)) ;
#10292=UNCERTAINTY_MEASURE_WITH_UNIT(LENGTH_MEASURE(0.001),#10335,
'DISTANCE_ACCURACY_VALUE',
'Maximum model space distance between geometric entities at asserted c
onnectivities') ;
#10297=UNCERTAINTY_MEASURE_WITH_UNIT(LENGTH_MEASURE(0.001),#10335,
'DISTANCE_ACCURACY_VALUE',
'Maximum model space distance between geometric entities at asserted c
onnectivities') ;
#10329=(
GEOMETRIC_REPRESENTATION_CONTEXT(3)
GLOBAL_UNCERTAINTY_ASSIGNED_CONTEXT((#10292))
GLOBAL_UNIT_ASSIGNED_CONTEXT((#10335,#10337,#10338))
REPRESENTATION_CONTEXT('','3D')
) ;
#10334=(
GEOMETRIC_REPRESENTATION_CONTEXT(3)
GLOBAL_UNCERTAINTY_ASSIGNED_CONTEXT((#10297))
GLOBAL_UNIT_ASSIGNED_CONTEXT((#10335,#10337,#10338))
REPRESENTATION_CONTEXT('','3D')
) ;
#10335=(
LENGTH_UNIT()
NAMED_UNIT(*)
SI_UNIT(.CENTI.,.METRE.)
) ;
#10337=(
NAMED_UNIT(*)
PLANE_ANGLE_UNIT()
SI_UNIT($,.RADIAN.)
) ;
#10338=(
NAMED_UNIT(*)
SI_UNIT($,.STERADIAN.)
SOLID_ANGLE_UNIT()
) ;
#10370=SHAPE_DEFINITION_REPRESENTATION(#10433,#10477) ;
#10433=PRODUCT_DEFINITION_SHAPE('',$,#10514) ;
#10477=SHAPE_REPRESENTATION('',(#4170),#10329) ;
#10482=PRODUCT_DEFINITION_CONTEXT('part definition',#10592,'design') ;
#10514=PRODUCT_DEFINITION('Mounting_Panel','Mounting_Panel',#10550,#10482) ;
#10550=PRODUCT_DEFINITION_FORMATION('',$,#10625) ;
#10592=APPLICATION_CONTEXT(
'Core Data for Automotive Mechanical Design Process') ;
#10593=PRODUCT_CONTEXT('part definition',#10592,'mechanical') ;
#10625=PRODUCT('Mounting_Panel','Mounting_Panel',$,(#10593)) ;
#10631=PRESENTATION_STYLE_ASSIGNMENT((#10635)) ;
#10635=SURFACE_STYLE_USAGE(.BOTH.,#10639) ;
#10639=SURFACE_SIDE_STYLE('',(#10643)) ;
#10643=SURFACE_STYLE_FILL_AREA(#10647) ;
#10647=FILL_AREA_STYLE('Opaque(25,25,25)',(#10651)) ;
#10651=FILL_AREA_STYLE_COLOUR('Opaque(25,25,25)',#10655) ;
#10655=COLOUR_RGB('Opaque(25,25,25)', 0.09019608, 0.27058824, 0.51372549) ;
ENDSEC;
END-ISO-10303-21;
